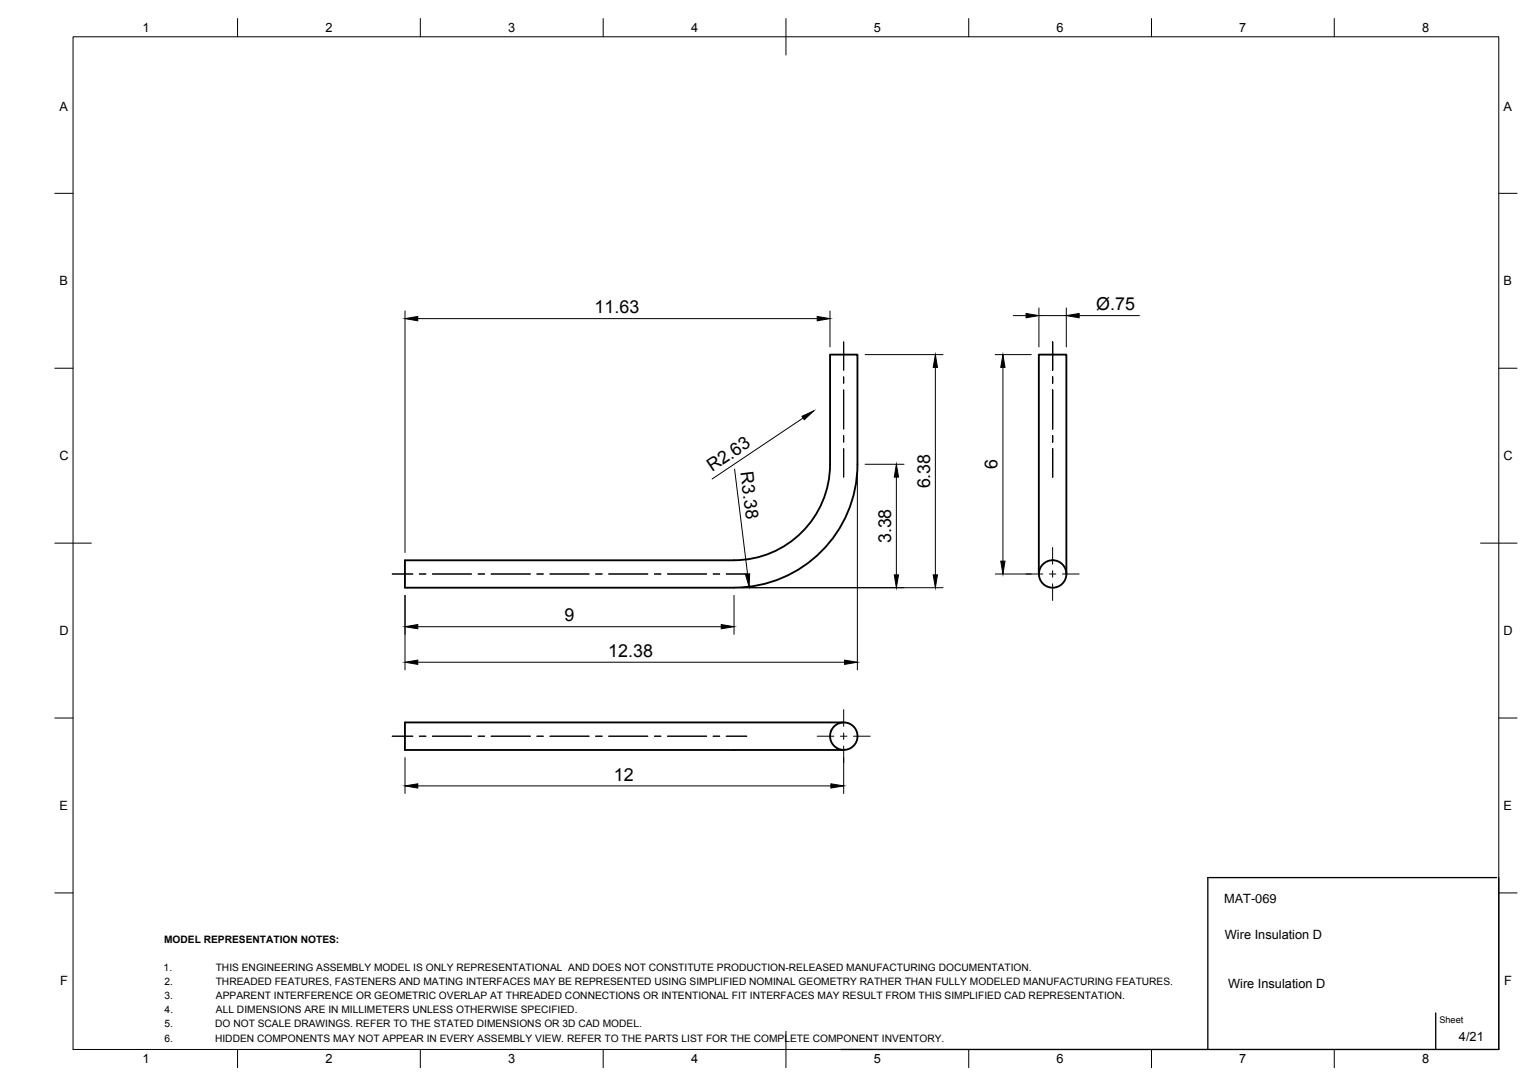
ISO-10303-21;
HEADER;
/* Generated by software containing ST-Developer
 * from STEP Tools, Inc. (www.steptools.com) 
 */

FILE_DESCRIPTION(
/* description */ ('CAx-IF Rec.Pracs.---Representation and Presentation of Product Manufa
cturing Information (PMI)---4.0---2014-10-13'),
/* implementation_level */ '2;1');

FILE_NAME(
/* name */ 'Wire Insulation D.step',
/* time_stamp */ '2026-10-24T15:08:39-07:00',
/* author */ (''),
/* organization */ (''),
/* preprocessor_version */ 'ST-DEVELOPER v20.2',
/* originating_system */ 'Autodesk Translation Framework v15.17.0.0',
/* authorisation */ '');

FILE_SCHEMA (('AP242_MANAGED_MODEL_BASED_3D_ENGINEERING_MIM_LF { 1 0 10303 442 2 1 4 }'));
ENDSEC;

DATA;
#10=MECHANICAL_DESIGN_GEOMETRIC_PRESENTATION_REPRESENTATION('',(#821),#50081);
#769=TOROIDAL_SURFACE('',#10120,0.003,0.000375);
#781=SHAPE_REPRESENTATION_RELATIONSHIP('SRR','None',#50149,#801);
#801=ADVANCED_BREP_SHAPE_REPRESENTATION('',(#841),#50062);
#821=STYLED_ITEM('',(#50258),#841);
#841=MANIFOLD_SOLID_BREP('Body1',#9866);
#862=PLANE('',#10114);
#863=PLANE('',#10125);
#1105=FACE_OUTER_BOUND('',#1646,.T.);
#1106=FACE_OUTER_BOUND('',#1647,.T.);
#1107=FACE_OUTER_BOUND('',#1648,.T.);
#1108=FACE_OUTER_BOUND('',#1649,.T.);
#1109=FACE_OUTER_BOUND('',#1650,.T.);
#1646=EDGE_LOOP('',(#6232));
#1647=EDGE_LOOP('',(#6233,#6234,#6235,#6236,#6237));
#1648=EDGE_LOOP('',(#6238,#6239,#6240,#6241,#6242,#6243));
#1649=EDGE_LOOP('',(#6244,#6245,#6246,#6247,#6248));
#1650=EDGE_LOOP('',(#6249));
#2244=LINE('',#13489,#2822);
#2245=LINE('',#13500,#2823);
#2822=VECTOR('',#11060,0.000375);
#2823=VECTOR('',#11075,0.000375);
#3401=CIRCLE('',#10115,0.00037500000001);
#3402=CIRCLE('',#10117,0.00037500000001);
#3403=CIRCLE('',#10118,0.00037500000001);
#3404=CIRCLE('',#10119,0.00037500000001);
#3405=CIRCLE('',#10121,0.002625);
#3406=CIRCLE('',#10122,0.00037500000001);
#3407=CIRCLE('',#10123,0.00037500000001);
#3774=VERTEX_POINT('',#13483);
#3775=VERTEX_POINT('',#13486);
#3776=VERTEX_POINT('',#13488);
#3777=VERTEX_POINT('',#13490);
#3778=VERTEX_POINT('',#13494);
#3779=VERTEX_POINT('',#13496);
#4769=EDGE_CURVE('',#3774,#3774,#3401,.T.);
#4770=EDGE_CURVE('',#3775,#3775,#3402,.T.);
#4771=EDGE_CURVE('',#3775,#3776,#2244,.T.);
#4772=EDGE_CURVE('',#3776,#3777,#3403,.T.);
#4773=EDGE_CURVE('',#3777,#3776,#3404,.T.);
#4774=EDGE_CURVE('',#3777,#3778,#3405,.T.);
#4775=EDGE_CURVE('',#3778,#3779,#3406,.T.);
#4776=EDGE_CURVE('',#3779,#3778,#3407,.T.);
#4777=EDGE_CURVE('',#3779,#3774,#2245,.T.);
#6232=ORIENTED_EDGE('',*,*,#4769,.F.);
#6233=ORIENTED_EDGE('',*,*,#4770,.F.);
#6234=ORIENTED_EDGE('',*,*,#4771,.T.);
#6235=ORIENTED_EDGE('',*,*,#4772,.T.);
#6236=ORIENTED_EDGE('',*,*,#4773,.T.);
#6237=ORIENTED_EDGE('',*,*,#4771,.F.);
#6238=ORIENTED_EDGE('',*,*,#4773,.F.);
#6239=ORIENTED_EDGE('',*,*,#4774,.T.);
#6240=ORIENTED_EDGE('',*,*,#4775,.T.);
#6241=ORIENTED_EDGE('',*,*,#4776,.T.);
#6242=ORIENTED_EDGE('',*,*,#4774,.F.);
#6243=ORIENTED_EDGE('',*,*,#4772,.F.);
#6244=ORIENTED_EDGE('',*,*,#4776,.F.);
#6245=ORIENTED_EDGE('',*,*,#4777,.T.);
#6246=ORIENTED_EDGE('',*,*,#4769,.T.);
#6247=ORIENTED_EDGE('',*,*,#4777,.F.);
#6248=ORIENTED_EDGE('',*,*,#4775,.F.);
#6249=ORIENTED_EDGE('',*,*,#4770,.T.);
#9147=CYLINDRICAL_SURFACE('',#10116,0.000375);
#9148=CYLINDRICAL_SURFACE('',#10124,0.000375);
#9327=ADVANCED_FACE('',(#1105),#862,.F.);
#9328=ADVANCED_FACE('',(#1106),#9147,.T.);
#9329=ADVANCED_FACE('',(#1107),#769,.T.);
#9330=ADVANCED_FACE('',(#1108),#9148,.T.);
#9331=ADVANCED_FACE('',(#1109),#863,.T.);
#9866=CLOSED_SHELL('',(#9327,#9328,#9329,#9330,#9331));
#10113=AXIS2_PLACEMENT_3D('',#13481,#11050,#11051);
#10114=AXIS2_PLACEMENT_3D('',#13482,#11052,#11053);
#10115=AXIS2_PLACEMENT_3D('',#13484,#11054,#11055);
#10116=AXIS2_PLACEMENT_3D('',#13485,#11056,#11057);
#10117=AXIS2_PLACEMENT_3D('',#13487,#11058,#11059);
#10118=AXIS2_PLACEMENT_3D('',#13491,#11061,#11062);
#10119=AXIS2_PLACEMENT_3D('',#13492,#11063,#11064);
#10120=AXIS2_PLACEMENT_3D('',#13493,#11065,#11066);
#10121=AXIS2_PLACEMENT_3D('',#13495,#11067,#11068);
#10122=AXIS2_PLACEMENT_3D('',#13497,#11069,#11070);
#10123=AXIS2_PLACEMENT_3D('',#13498,#11071,#11072);
#10124=AXIS2_PLACEMENT_3D('',#13499,#11073,#11074);
#10125=AXIS2_PLACEMENT_3D('',#13501,#11076,#11077);
#11050=DIRECTION('axis',(0.,0.,1.));
#11051=DIRECTION('refdir',(1.,0.,0.));
#11052=DIRECTION('center_axis',(0.906307787036647,-0.422618261740706,-8.00429517722823E-16));
#11053=DIRECTION('ref_axis',(2.42833204006769E-16,2.41473507855972E-15,
-1.));
#11054=DIRECTION('center_axis',(0.906307787036647,-0.422618261740706,-8.00429517722823E-16));
#11055=DIRECTION('ref_axis',(0.422618261740706,0.906307787036647,1.97116866169388E-15));
#11056=DIRECTION('center_axis',(2.42833204006769E-16,2.41473507855972E-15,
-1.));
#11057=DIRECTION('ref_axis',(0.422618261740706,0.906307787036647,2.29111895189949E-15));
#11058=DIRECTION('center_axis',(2.41685059822166E-11,-1.12674314556115E-11,
-1.));
#11059=DIRECTION('ref_axis',(0.422618261740706,0.906307787036647,2.29111895186703E-15));
#11060=DIRECTION('',(-2.42833204006769E-16,-2.41473507855972E-15,1.));
#11061=DIRECTION('center_axis',(2.41685059822166E-11,-1.12674314556115E-11,
-1.));
#11062=DIRECTION('ref_axis',(0.422618261740706,0.906307787036647,2.29111895186703E-15));
#11063=DIRECTION('center_axis',(2.41685059822166E-11,-1.12674314556115E-11,
-1.));
#11064=DIRECTION('ref_axis',(0.422618261740706,0.906307787036647,2.29111895186703E-15));
#11065=DIRECTION('center_axis',(0.422618261740706,0.906307787036647,1.97116866169388E-15));
#11066=DIRECTION('ref_axis',(1.28498035257541E-16,2.05596856412066E-15,
-1.));
#11067=DIRECTION('center_axis',(-0.422618261740706,-0.906307787036647,-1.97116866169388E-15));
#11068=DIRECTION('ref_axis',(3.58767987664542E-16,2.00764771571504E-15,
-1.));
#11069=DIRECTION('center_axis',(0.906307787036647,-0.422618261740706,-8.00429517722823E-16));
#11070=DIRECTION('ref_axis',(0.422618261740706,0.906307787036647,1.97116866169388E-15));
#11071=DIRECTION('center_axis',(0.906307787036647,-0.422618261740706,-8.00429517722823E-16));
#11072=DIRECTION('ref_axis',(0.422618261740706,0.906307787036647,1.97116866169388E-15));
#11073=DIRECTION('center_axis',(0.906307787036647,-0.422618261740706,-8.00429517722823E-16));
#11074=DIRECTION('ref_axis',(0.422618261740706,0.906307787036647,1.97116866169388E-15));
#11075=DIRECTION('',(-0.906307787036647,0.422618261740706,8.00429517722823E-16));
#11076=DIRECTION('center_axis',(2.98328550528607E-16,2.38885717348462E-15,
-1.));
#11077=DIRECTION('ref_axis',(0.906307787036647,-0.422618261740706,-7.39197177765454E-16));
#13481=CARTESIAN_POINT('',(0.,0.,0.));
#13482=CARTESIAN_POINT('Origin',(-0.00508700257531012,-0.0309105091425022,
0.0016241467134419));
#13483=CARTESIAN_POINT('',(-0.0052454844234719,-0.0312503745626367,0.0016241467134419));
#13484=CARTESIAN_POINT('Origin',(-0.00508700257532341,-0.0309105091425071,
0.0016241467134519));
#13485=CARTESIAN_POINT('Origin',(0.00578869086912964,-0.0359819282833906,
-0.0013758532865581));
#13486=CARTESIAN_POINT('',(0.00563020902097688,-0.0363217937035293,-0.0043758532865581));
#13487=CARTESIAN_POINT('Origin',(0.00578869086912542,-0.0359819282833998,
-0.0043758532865481));
#13488=CARTESIAN_POINT('',(0.00563020902097688,-0.0363217937035293,-0.0013758532865381));
#13489=CARTESIAN_POINT('',(0.00563020902097688,-0.0363217937035293,-0.0013758532865581));
#13490=CARTESIAN_POINT('',(0.00544882544898185,-0.0358234464352337,-0.0013758532865581));
#13491=CARTESIAN_POINT('Origin',(0.00578869086912542,-0.0359819282833998,
-0.0013758532865481));
#13492=CARTESIAN_POINT('Origin',(0.00578869086912542,-0.0359819282833998,
-0.0013758532865481));
#13493=CARTESIAN_POINT('Origin',(0.0030697675080197,-0.0347140734981686,
-0.0013758532865581));
#13494=CARTESIAN_POINT('',(0.00306976750801062,-0.0347140734981644,0.0012491467134419));
#13495=CARTESIAN_POINT('Origin',(0.0030697675080197,-0.0347140734981686,
-0.0013758532865581));
#13496=CARTESIAN_POINT('',(0.00291128565985791,-0.035053938918303,0.0016241467134419));
#13497=CARTESIAN_POINT('Origin',(0.00306976750800641,-0.0347140734981734,
0.0016241467134519));
#13498=CARTESIAN_POINT('Origin',(0.00306976750800641,-0.0347140734981734,
0.0016241467134519));
#13499=CARTESIAN_POINT('Origin',(-0.01052484929753,-0.0283747995720579,
0.00162414671344191));
#13500=CARTESIAN_POINT('',(-0.0106833311456828,-0.0287146649921966,0.00162414671344191));
#13501=CARTESIAN_POINT('Origin',(0.00578869086912964,-0.0359819282833906,
-0.0043758532865581));
#50040=UNCERTAINTY_MEASURE_WITH_UNIT(LENGTH_MEASURE(1.E-5),#50082,
'DISTANCE_ACCURACY_VALUE',
'Maximum model space distance between geometric entities at asserted c
onnectivities');
#50059=UNCERTAINTY_MEASURE_WITH_UNIT(LENGTH_MEASURE(1.E-5),#50082,
'DISTANCE_ACCURACY_VALUE',
'Maximum model space distance between geometric entities at asserted c
onnectivities');
#50062=(
GEOMETRIC_REPRESENTATION_CONTEXT(3)
GLOBAL_UNCERTAINTY_ASSIGNED_CONTEXT((#50040))
GLOBAL_UNIT_ASSIGNED_CONTEXT((#50082,#50083,#50084))
REPRESENTATION_CONTEXT('','3D')
);
#50081=(
GEOMETRIC_REPRESENTATION_CONTEXT(3)
GLOBAL_UNCERTAINTY_ASSIGNED_CONTEXT((#50059))
GLOBAL_UNIT_ASSIGNED_CONTEXT((#50082,#50083,#50084))
REPRESENTATION_CONTEXT('','3D')
);
#50082=(
LENGTH_UNIT()
NAMED_UNIT(*)
SI_UNIT($,.METRE.)
);
#50083=(
NAMED_UNIT(*)
PLANE_ANGLE_UNIT()
SI_UNIT($,.RADIAN.)
);
#50084=(
NAMED_UNIT(*)
SI_UNIT($,.STERADIAN.)
SOLID_ANGLE_UNIT()
);
#50087=SHAPE_DEFINITION_REPRESENTATION(#50108,#50149);
#50108=PRODUCT_DEFINITION_SHAPE('',$,#50171);
#50149=SHAPE_REPRESENTATION('',(#10113),#50062);
#50168=PRODUCT_DEFINITION_CONTEXT('part definition',#50233,'design');
#50171=PRODUCT_DEFINITION('Wire Insulation D','Wire Insulation D',#50192,
#50168);
#50192=PRODUCT_DEFINITION_FORMATION('',$,#50237);
#50233=APPLICATION_CONTEXT('Managed model based 3d engineering');
#50234=PRODUCT_CONTEXT('part definition',#50233,'mechanical');
#50237=PRODUCT('Wire Insulation D','Wire Insulation D',
'LEGAL AND USAGE DISCLAIMER: this Data/Model is provided \X2\201C\X0\A
S IS\X2\201D\X0\ for informational and representational only. It is a 
geometric approximation and is NOT engineered, certified, or guarantee
d for dimensional accuracy, exact tolerances, or production-level prec
ision. Vendor disclaims all implied warranties including fitness for a
 particular purpose. DO NOT USE FOR DIRECT PHYSICAL MANUFACTURING, AUT
OMATED PRODUCTION, OR SAFETY-CRITICAL SYSTEMS without independent engi
neering verification and resolution of any design discrepancies.',(#50234));
#50258=PRESENTATION_STYLE_ASSIGNMENT((#50265));
#50265=SURFACE_STYLE_USAGE(.BOTH.,#50272);
#50272=SURFACE_SIDE_STYLE('',(#50279));
#50279=SURFACE_STYLE_FILL_AREA(#50286);
#50286=FILL_AREA_STYLE('Opaque(89,149,218)',(#50293));
#50293=FILL_AREA_STYLE_COLOUR('Opaque(89,149,218)',#50300);
#50300=COLOUR_RGB('Opaque(89,149,218)',0.349019607843137,0.584313725490196,
0.854901960784314);
ENDSEC;
END-ISO-10303-21;
